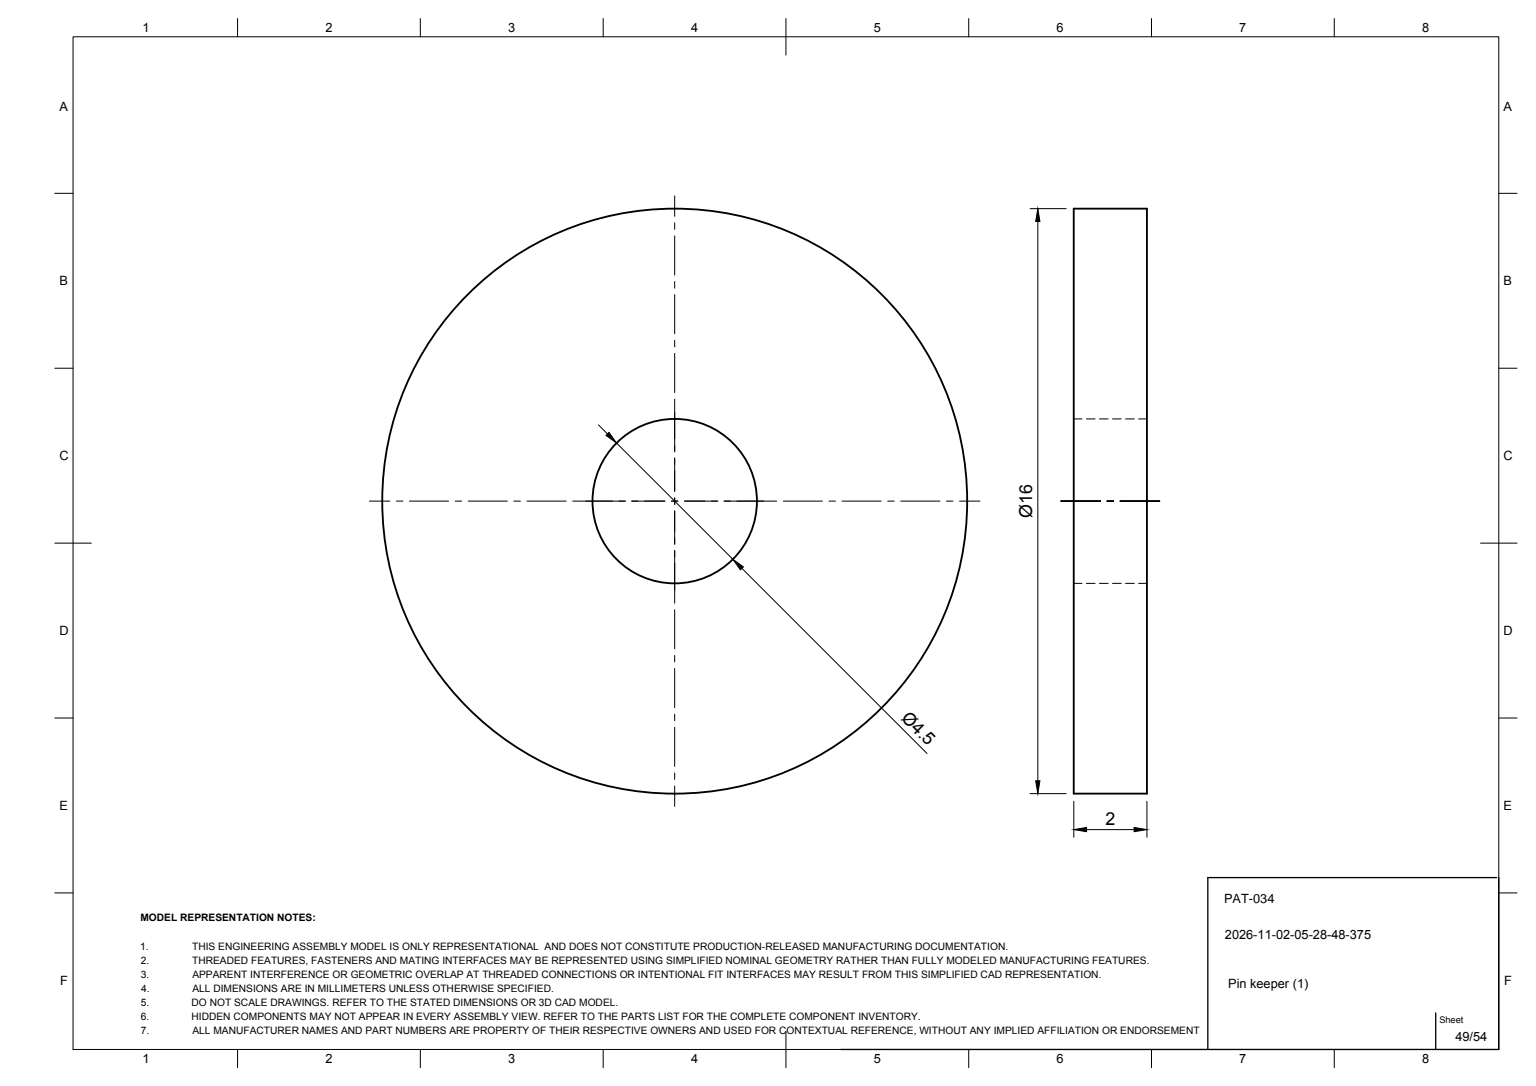
ISO-10303-21;
HEADER;
/* Generated by software containing ST-Developer
 * from STEP Tools, Inc. (www.steptools.com) 
 */

FILE_DESCRIPTION(
/* description */ ('Fatigue rig crank-slider'),
/* implementation_level */ '2;1');

FILE_NAME(
/* name */ 'Pin keeper (1).step',
/* time_stamp */ '2026-10-28T03:24:50-07:00',
/* author */ (''),
/* organization */ (''),
/* preprocessor_version */ 'ST-DEVELOPER v20.2',
/* originating_system */ 'Autodesk Translation Framework v15.17.0.0',
/* authorisation */ '');

FILE_SCHEMA (('AUTOMOTIVE_DESIGN { 1 0 10303 214 3 1 1 }'));
ENDSEC;

DATA;
#10=MECHANICAL_DESIGN_GEOMETRIC_PRESENTATION_REPRESENTATION('',(#638),#16911);
#529=SHAPE_REPRESENTATION_RELATIONSHIP('SRR','None',#17173,#579);
#579=ADVANCED_BREP_SHAPE_REPRESENTATION('',(#695),#16902);
#638=STYLED_ITEM('',(#17487),#695);
#695=MANIFOLD_SOLID_BREP('Body1',#8931);
#886=FACE_BOUND('',#2352,.T.);
#887=FACE_BOUND('',#2354,.T.);
#1142=PLANE('',#10339);
#1143=PLANE('',#10340);
#1640=FACE_OUTER_BOUND('',#2349,.T.);
#1641=FACE_OUTER_BOUND('',#2350,.T.);
#1642=FACE_OUTER_BOUND('',#2351,.T.);
#1643=FACE_OUTER_BOUND('',#2353,.T.);
#2349=EDGE_LOOP('',(#7744,#7745,#7746,#7747));
#2350=EDGE_LOOP('',(#7748,#7749,#7750,#7751));
#2351=EDGE_LOOP('',(#7752));
#2352=EDGE_LOOP('',(#7753));
#2353=EDGE_LOOP('',(#7754));
#2354=EDGE_LOOP('',(#7755));
#2927=LINE('',#16239,#3573);
#2928=LINE('',#16245,#3574);
#3573=VECTOR('',#12717,0.225);
#3574=VECTOR('',#12724,0.800000000000001);
#4105=CIRCLE('',#10334,0.225);
#4106=CIRCLE('',#10335,0.225);
#4107=CIRCLE('',#10337,0.800000000000001);
#4108=CIRCLE('',#10338,0.800000000000001);
#4749=VERTEX_POINT('',#16236);
#4750=VERTEX_POINT('',#16238);
#4751=VERTEX_POINT('',#16242);
#4752=VERTEX_POINT('',#16244);
#5770=EDGE_CURVE('',#4749,#4749,#4105,.T.);
#5771=EDGE_CURVE('',#4749,#4750,#2927,.T.);
#5772=EDGE_CURVE('',#4750,#4750,#4106,.T.);
#5773=EDGE_CURVE('',#4751,#4751,#4107,.T.);
#5774=EDGE_CURVE('',#4751,#4752,#2928,.T.);
#5775=EDGE_CURVE('',#4752,#4752,#4108,.T.);
#7744=ORIENTED_EDGE('',*,*,#5770,.F.);
#7745=ORIENTED_EDGE('',*,*,#5771,.T.);
#7746=ORIENTED_EDGE('',*,*,#5772,.T.);
#7747=ORIENTED_EDGE('',*,*,#5771,.F.);
#7748=ORIENTED_EDGE('',*,*,#5773,.F.);
#7749=ORIENTED_EDGE('',*,*,#5774,.T.);
#7750=ORIENTED_EDGE('',*,*,#5775,.T.);
#7751=ORIENTED_EDGE('',*,*,#5774,.F.);
#7752=ORIENTED_EDGE('',*,*,#5773,.T.);
#7753=ORIENTED_EDGE('',*,*,#5770,.T.);
#7754=ORIENTED_EDGE('',*,*,#5775,.F.);
#7755=ORIENTED_EDGE('',*,*,#5772,.F.);
#8341=CYLINDRICAL_SURFACE('',#10333,0.225);
#8342=CYLINDRICAL_SURFACE('',#10336,0.800000000000001);
#8778=ADVANCED_FACE('',(#1640),#8341,.F.);
#8779=ADVANCED_FACE('',(#1641),#8342,.T.);
#8780=ADVANCED_FACE('',(#1642,#886),#1142,.T.);
#8781=ADVANCED_FACE('',(#1643,#887),#1143,.F.);
#8931=CLOSED_SHELL('',(#8778,#8779,#8780,#8781));
#10332=AXIS2_PLACEMENT_3D('',#16234,#12711,#12712);
#10333=AXIS2_PLACEMENT_3D('',#16235,#12713,#12714);
#10334=AXIS2_PLACEMENT_3D('',#16237,#12715,#12716);
#10335=AXIS2_PLACEMENT_3D('',#16240,#12718,#12719);
#10336=AXIS2_PLACEMENT_3D('',#16241,#12720,#12721);
#10337=AXIS2_PLACEMENT_3D('',#16243,#12722,#12723);
#10338=AXIS2_PLACEMENT_3D('',#16246,#12725,#12726);
#10339=AXIS2_PLACEMENT_3D('',#16247,#12727,#12728);
#10340=AXIS2_PLACEMENT_3D('',#16248,#12729,#12730);
#12711=DIRECTION('axis',(0.,0.,1.));
#12712=DIRECTION('refdir',(1.,0.,0.));
#12713=DIRECTION('center_axis',(0.,1.,0.));
#12714=DIRECTION('ref_axis',(1.,0.,0.));
#12715=DIRECTION('center_axis',(0.,-1.,0.));
#12716=DIRECTION('ref_axis',(1.,0.,0.));
#12717=DIRECTION('',(0.,-1.,0.));
#12718=DIRECTION('center_axis',(0.,-1.,0.));
#12719=DIRECTION('ref_axis',(1.,0.,0.));
#12720=DIRECTION('center_axis',(0.,1.,0.));
#12721=DIRECTION('ref_axis',(1.,0.,0.));
#12722=DIRECTION('center_axis',(0.,1.,0.));
#12723=DIRECTION('ref_axis',(1.,0.,0.));
#12724=DIRECTION('',(0.,-1.,0.));
#12725=DIRECTION('center_axis',(0.,1.,0.));
#12726=DIRECTION('ref_axis',(1.,0.,0.));
#12727=DIRECTION('center_axis',(0.,1.,0.));
#12728=DIRECTION('ref_axis',(1.,0.,0.));
#12729=DIRECTION('center_axis',(0.,1.,0.));
#12730=DIRECTION('ref_axis',(1.,0.,0.));
#16234=CARTESIAN_POINT('',(0.,0.,0.));
#16235=CARTESIAN_POINT('Origin',(11.,4.8,12.));
#16236=CARTESIAN_POINT('',(10.775,5.,12.));
#16237=CARTESIAN_POINT('Origin',(11.,5.,12.));
#16238=CARTESIAN_POINT('',(10.775,4.8,12.));
#16239=CARTESIAN_POINT('',(10.775,4.8,12.));
#16240=CARTESIAN_POINT('Origin',(11.,4.8,12.));
#16241=CARTESIAN_POINT('Origin',(11.,4.8,12.));
#16242=CARTESIAN_POINT('',(10.2,5.,12.));
#16243=CARTESIAN_POINT('Origin',(11.,5.,12.));
#16244=CARTESIAN_POINT('',(10.2,4.8,12.));
#16245=CARTESIAN_POINT('',(10.2,4.8,12.));
#16246=CARTESIAN_POINT('Origin',(11.,4.8,12.));
#16247=CARTESIAN_POINT('Origin',(11.,5.,12.));
#16248=CARTESIAN_POINT('Origin',(11.,4.8,12.));
#16843=UNCERTAINTY_MEASURE_WITH_UNIT(LENGTH_MEASURE(0.001),#16912,
'DISTANCE_ACCURACY_VALUE',
'Maximum model space distance between geometric entities at asserted c
onnectivities');
#16852=UNCERTAINTY_MEASURE_WITH_UNIT(LENGTH_MEASURE(0.001),#16912,
'DISTANCE_ACCURACY_VALUE',
'Maximum model space distance between geometric entities at asserted c
onnectivities');
#16902=(
GEOMETRIC_REPRESENTATION_CONTEXT(3)
GLOBAL_UNCERTAINTY_ASSIGNED_CONTEXT((#16843))
GLOBAL_UNIT_ASSIGNED_CONTEXT((#16912,#16914,#16915))
REPRESENTATION_CONTEXT('','3D')
);
#16911=(
GEOMETRIC_REPRESENTATION_CONTEXT(3)
GLOBAL_UNCERTAINTY_ASSIGNED_CONTEXT((#16852))
GLOBAL_UNIT_ASSIGNED_CONTEXT((#16912,#16914,#16915))
REPRESENTATION_CONTEXT('','3D')
);
#16912=(
LENGTH_UNIT()
NAMED_UNIT(*)
SI_UNIT(.CENTI.,.METRE.)
);
#16914=(
NAMED_UNIT(*)
PLANE_ANGLE_UNIT()
SI_UNIT($,.RADIAN.)
);
#16915=(
NAMED_UNIT(*)
SI_UNIT($,.STERADIAN.)
SOLID_ANGLE_UNIT()
);
#16965=SHAPE_DEFINITION_REPRESENTATION(#17037,#17173);
#17037=PRODUCT_DEFINITION_SHAPE('',$,#17232);
#17173=SHAPE_REPRESENTATION('',(#10332),#16902);
#17182=PRODUCT_DEFINITION_CONTEXT('part definition',#17358,'design');
#17232=PRODUCT_DEFINITION('Pin keeper (1)','Pin keeper (1)',#17290,#17182);
#17290=PRODUCT_DEFINITION_FORMATION('',$,#17409);
#17358=APPLICATION_CONTEXT(
'Core Data for Automotive Mechanical Design Process');
#17359=PRODUCT_CONTEXT('part definition',#17358,'mechanical');
#17409=PRODUCT('Pin keeper (1)','Pin keeper (1)','Pin keeper (1)',(#17359));
#17481=COLOUR_RGB('Grey',0.48,0.52,0.57);
#17482=FILL_AREA_STYLE_COLOUR('',#17481);
#17483=FILL_AREA_STYLE('',(#17482));
#17484=SURFACE_STYLE_FILL_AREA(#17483);
#17485=SURFACE_SIDE_STYLE('',(#17484));
#17486=SURFACE_STYLE_USAGE(.BOTH.,#17485);
#17487=PRESENTATION_STYLE_ASSIGNMENT((#17486));
ENDSEC;
END-ISO-10303-21;
